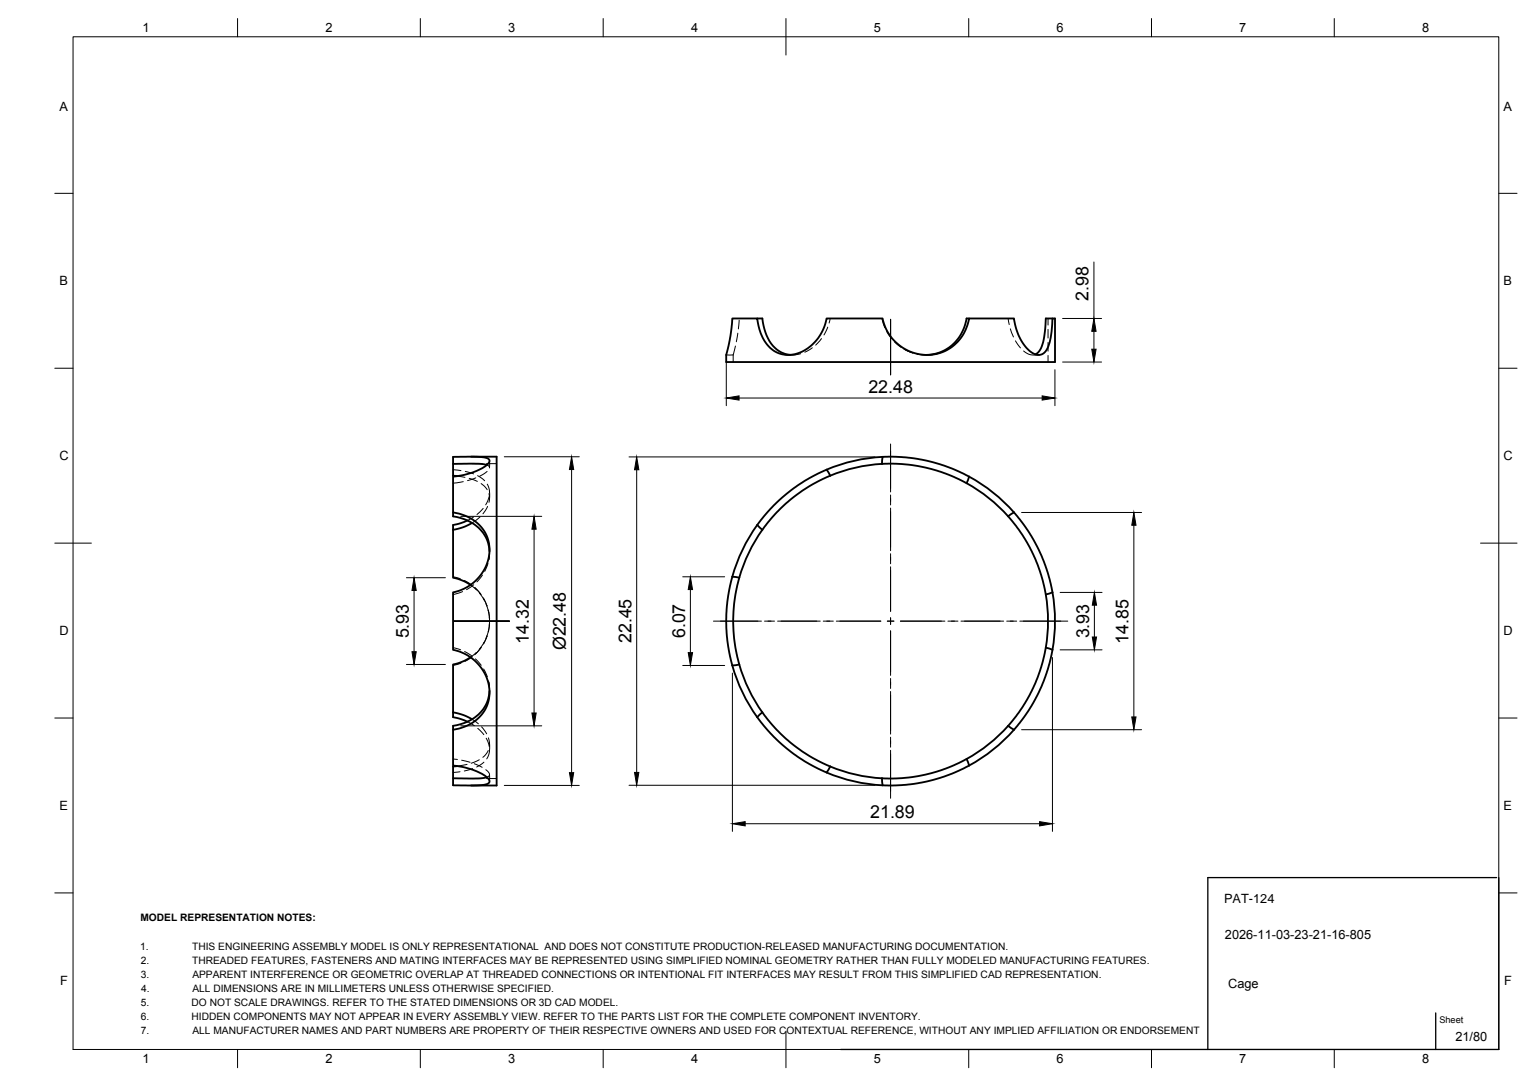
ISO-10303-21;
HEADER;
/* Generated by software containing ST-Developer
 * from STEP Tools, Inc. (www.steptools.com) 
 */

FILE_DESCRIPTION(
/* description */ ('XY cross-slide table'),
/* implementation_level */ '2;1');

FILE_NAME(
/* name */ 'Cage.step',
/* time_stamp */ '2026-10-28T03:22:46-07:00',
/* author */ (''),
/* organization */ (''),
/* preprocessor_version */ 'ST-DEVELOPER v20.2',
/* originating_system */ 'Autodesk Translation Framework v15.17.0.0',
/* authorisation */ '');

FILE_SCHEMA (('AUTOMOTIVE_DESIGN { 1 0 10303 214 3 1 1 }'));
ENDSEC;

DATA;
#10=MECHANICAL_DESIGN_GEOMETRIC_PRESENTATION_REPRESENTATION('',(#1690),#62984);
#693=B_SPLINE_CURVE_WITH_KNOTS('',3,(#33674,#33675,#33676,#33677,#33678,
#33679,#33680,#33681,#33682,#33683,#33684,#33685,#33686,#33687,#33688,#33689,
#33690,#33691,#33692,#33693,#33694,#33695),.UNSPECIFIED.,.F.,.F.,(4,2,2,
2,2,2,2,2,2,2,4),(0.0591825211272536,0.157966726598481,0.236950089897721,
0.315933453196962,0.391576304923761,0.46721915665056,0.54286200837736,0.618504860104159,
0.697488223403399,0.77647158670264,0.875255792173867),.UNSPECIFIED.);
#694=B_SPLINE_CURVE_WITH_KNOTS('',3,(#33699,#33700,#33701,#33702,#33703,
#33704,#33705,#33706,#33707,#33708,#33709,#33710,#33711,#33712,#33713,#33714,
#33715,#33716,#33717,#33718,#33719,#33720),.UNSPECIFIED.,.F.,.F.,(4,2,2,
2,2,2,2,2,2,2,4),(0.0581119756758434,0.106553146291161,0.213106292582322,
0.30849933801665,0.386091982889075,0.4636846277615,0.541277272633925,0.61886991750635,
0.714262962940678,0.820816109231839,0.869257279847157),.UNSPECIFIED.);
#695=B_SPLINE_CURVE_WITH_KNOTS('',3,(#33726,#33727,#33728,#33729,#33730,
#33731,#33732,#33733,#33734,#33735,#33736,#33737,#33738,#33739,#33740,#33741,
#33742,#33743,#33744,#33745,#33746,#33747),.UNSPECIFIED.,.F.,.F.,(4,2,2,
2,2,2,2,2,2,2,4),(0.0581119756758434,0.106553146291161,0.213106292582322,
0.30849933801665,0.386091982889075,0.4636846277615,0.541277272633925,0.61886991750635,
0.714262962940679,0.820816109231839,0.869257279847157),.UNSPECIFIED.);
#696=B_SPLINE_CURVE_WITH_KNOTS('',3,(#33751,#33752,#33753,#33754,#33755,
#33756,#33757,#33758,#33759,#33760,#33761,#33762,#33763,#33764,#33765,#33766,
#33767,#33768,#33769,#33770,#33771,#33772),.UNSPECIFIED.,.F.,.F.,(4,2,2,
2,2,2,2,2,2,2,4),(0.0581119756758433,0.106553146291161,0.213106292582322,
0.308499338016649,0.386091982889075,0.4636846277615,0.541277272633925,0.61886991750635,
0.714262962940678,0.820816109231839,0.869257279847157),.UNSPECIFIED.);
#697=B_SPLINE_CURVE_WITH_KNOTS('',3,(#33781,#33782,#33783,#33784,#33785,
#33786,#33787,#33788,#33789,#33790,#33791,#33792,#33793,#33794,#33795,#33796,
#33797,#33798,#33799,#33800,#33801,#33802),.UNSPECIFIED.,.F.,.F.,(4,2,2,
2,2,2,2,2,2,2,4),(0.0581119756758433,0.106553146291161,0.213106292582322,
0.30849933801665,0.386091982889075,0.4636846277615,0.541277272633925,0.61886991750635,
0.714262962940678,0.820816109231839,0.869257279847157),.UNSPECIFIED.);
#698=B_SPLINE_CURVE_WITH_KNOTS('',3,(#33806,#33807,#33808,#33809,#33810,
#33811,#33812,#33813,#33814,#33815,#33816,#33817,#33818,#33819,#33820,#33821,
#33822,#33823,#33824,#33825,#33826,#33827),.UNSPECIFIED.,.F.,.F.,(4,2,2,
2,2,2,2,2,2,2,4),(0.0581119756758434,0.106553146291161,0.213106292582322,
0.30849933801665,0.386091982889075,0.4636846277615,0.541277272633925,0.61886991750635,
0.714262962940678,0.820816109231839,0.869257279847157),.UNSPECIFIED.);
#699=B_SPLINE_CURVE_WITH_KNOTS('',3,(#33831,#33832,#33833,#33834,#33835,
#33836,#33837,#33838,#33839,#33840,#33841,#33842,#33843,#33844,#33845,#33846,
#33847,#33848,#33849,#33850,#33851,#33852),.UNSPECIFIED.,.F.,.F.,(4,2,2,
2,2,2,2,2,2,2,4),(0.0581119756758434,0.106553146291161,0.213106292582322,
0.30849933801665,0.386091982889075,0.4636846277615,0.541277272633925,0.61886991750635,
0.714262962940678,0.820816109231839,0.869257279847157),.UNSPECIFIED.);
#700=B_SPLINE_CURVE_WITH_KNOTS('',3,(#33856,#33857,#33858,#33859,#33860,
#33861,#33862,#33863,#33864,#33865,#33866,#33867,#33868,#33869,#33870,#33871,
#33872,#33873,#33874,#33875,#33876,#33877),.UNSPECIFIED.,.F.,.F.,(4,2,2,
2,2,2,2,2,2,2,4),(0.0581119756758433,0.106553146291161,0.213106292582322,
0.30849933801665,0.386091982889075,0.4636846277615,0.541277272633925,0.61886991750635,
0.714262962940678,0.820816109231839,0.869257279847157),.UNSPECIFIED.);
#701=B_SPLINE_CURVE_WITH_KNOTS('',3,(#33885,#33886,#33887,#33888,#33889,
#33890,#33891,#33892,#33893,#33894,#33895,#33896,#33897,#33898,#33899,#33900,
#33901,#33902,#33903,#33904,#33905,#33906),.UNSPECIFIED.,.F.,.F.,(4,2,2,
2,2,2,2,2,2,2,4),(0.0591825211272536,0.157966726598481,0.236950089897721,
0.315933453196962,0.391576304923761,0.467219156650561,0.54286200837736,
0.618504860104159,0.697488223403399,0.77647158670264,0.875255792173867),
 .UNSPECIFIED.);
#702=B_SPLINE_CURVE_WITH_KNOTS('',3,(#33914,#33915,#33916,#33917,#33918,
#33919,#33920,#33921,#33922,#33923,#33924,#33925,#33926,#33927,#33928,#33929,
#33930,#33931,#33932,#33933,#33934,#33935),.UNSPECIFIED.,.F.,.F.,(4,2,2,
2,2,2,2,2,2,2,4),(0.0591825211272536,0.157966726598481,0.236950089897722,
0.315933453196962,0.391576304923761,0.467219156650561,0.54286200837736,
0.618504860104159,0.697488223403399,0.77647158670264,0.875255792173867),
 .UNSPECIFIED.);
#703=B_SPLINE_CURVE_WITH_KNOTS('',3,(#33945,#33946,#33947,#33948,#33949,
#33950,#33951,#33952,#33953,#33954,#33955,#33956,#33957,#33958,#33959,#33960,
#33961,#33962,#33963,#33964,#33965,#33966),.UNSPECIFIED.,.F.,.F.,(4,2,2,
2,2,2,2,2,2,2,4),(0.0591825211272536,0.157966726598481,0.236950089897721,
0.315933453196962,0.391576304923761,0.46721915665056,0.54286200837736,0.618504860104159,
0.697488223403399,0.77647158670264,0.875255792173867),.UNSPECIFIED.);
#704=B_SPLINE_CURVE_WITH_KNOTS('',3,(#33974,#33975,#33976,#33977,#33978,
#33979,#33980,#33981,#33982,#33983,#33984,#33985,#33986,#33987,#33988,#33989,
#33990,#33991,#33992,#33993,#33994,#33995),.UNSPECIFIED.,.F.,.F.,(4,2,2,
2,2,2,2,2,2,2,4),(0.0591825211272536,0.157966726598481,0.236950089897721,
0.315933453196962,0.391576304923761,0.46721915665056,0.542862008377359,
0.618504860104159,0.697488223403399,0.776471586702639,0.875255792173867),
 .UNSPECIFIED.);
#705=B_SPLINE_CURVE_WITH_KNOTS('',3,(#34003,#34004,#34005,#34006,#34007,
#34008,#34009,#34010,#34011,#34012,#34013,#34014,#34015,#34016,#34017,#34018,
#34019,#34020,#34021,#34022,#34023,#34024),.UNSPECIFIED.,.F.,.F.,(4,2,2,
2,2,2,2,2,2,2,4),(0.0591825211272536,0.157966726598481,0.236950089897721,
0.315933453196962,0.391576304923761,0.46721915665056,0.54286200837736,0.618504860104159,
0.697488223403399,0.77647158670264,0.875255792173867),.UNSPECIFIED.);
#706=B_SPLINE_CURVE_WITH_KNOTS('',3,(#34033,#34034,#34035,#34036,#34037,
#34038,#34039,#34040,#34041,#34042,#34043,#34044,#34045,#34046,#34047,#34048,
#34049,#34050,#34051,#34052,#34053,#34054),.UNSPECIFIED.,.F.,.F.,(4,2,2,
2,2,2,2,2,2,2,4),(0.0591825211272536,0.157966726598481,0.236950089897721,
0.315933453196962,0.391576304923761,0.46721915665056,0.542862008377359,
0.618504860104159,0.697488223403399,0.776471586702639,0.875255792173867),
 .UNSPECIFIED.);
#1388=SPHERICAL_SURFACE('',#24342,0.309556);
#1389=SPHERICAL_SURFACE('',#24358,0.309556);
#1390=SPHERICAL_SURFACE('',#24363,0.309556);
#1391=SPHERICAL_SURFACE('',#24369,0.309556);
#1392=SPHERICAL_SURFACE('',#24374,0.309556);
#1393=SPHERICAL_SURFACE('',#24379,0.309556);
#1394=SPHERICAL_SURFACE('',#24387,0.309556);
#1518=SHAPE_REPRESENTATION_RELATIONSHIP('SRR','None',#63367,#1601);
#1601=ADVANCED_BREP_SHAPE_REPRESENTATION('',(#1803),#62904);
#1690=STYLED_ITEM('',(#63912),#1803);
#1803=MANIFOLD_SOLID_BREP('Continuous crown cage',#22984);
#1987=FACE_BOUND('',#4469,.T.);
#2385=PLANE('',#24355);
#2386=PLANE('',#24360);
#2387=PLANE('',#24365);
#2388=PLANE('',#24371);
#2389=PLANE('',#24376);
#2390=PLANE('',#24385);
#2391=PLANE('',#24389);
#2392=PLANE('',#24390);
#3039=FACE_OUTER_BOUND('',#4453,.T.);
#3040=FACE_OUTER_BOUND('',#4454,.T.);
#3041=FACE_OUTER_BOUND('',#4455,.T.);
#3042=FACE_OUTER_BOUND('',#4456,.T.);
#3043=FACE_OUTER_BOUND('',#4457,.T.);
#3044=FACE_OUTER_BOUND('',#4458,.T.);
#3045=FACE_OUTER_BOUND('',#4459,.T.);
#3046=FACE_OUTER_BOUND('',#4460,.T.);
#3047=FACE_OUTER_BOUND('',#4461,.T.);
#3048=FACE_OUTER_BOUND('',#4462,.T.);
#3049=FACE_OUTER_BOUND('',#4463,.T.);
#3050=FACE_OUTER_BOUND('',#4464,.T.);
#3051=FACE_OUTER_BOUND('',#4465,.T.);
#3052=FACE_OUTER_BOUND('',#4466,.T.);
#3053=FACE_OUTER_BOUND('',#4467,.T.);
#3054=FACE_OUTER_BOUND('',#4468,.T.);
#3055=FACE_OUTER_BOUND('',#4470,.T.);
#4453=EDGE_LOOP('',(#15632,#15633,#15634,#15635));
#4454=EDGE_LOOP('',(#15636,#15637,#15638,#15639,#15640,#15641,#15642,#15643,
#15644,#15645,#15646,#15647,#15648,#15649,#15650,#15651,#15652,#15653));
#4455=EDGE_LOOP('',(#15654,#15655,#15656,#15657));
#4456=EDGE_LOOP('',(#15658,#15659,#15660,#15661));
#4457=EDGE_LOOP('',(#15662,#15663,#15664,#15665));
#4458=EDGE_LOOP('',(#15666,#15667,#15668,#15669));
#4459=EDGE_LOOP('',(#15670,#15671,#15672,#15673,#15674,#15675));
#4460=EDGE_LOOP('',(#15676,#15677,#15678,#15679));
#4461=EDGE_LOOP('',(#15680,#15681,#15682,#15683));
#4462=EDGE_LOOP('',(#15684,#15685,#15686,#15687));
#4463=EDGE_LOOP('',(#15688,#15689,#15690,#15691));
#4464=EDGE_LOOP('',(#15692,#15693,#15694,#15695));
#4465=EDGE_LOOP('',(#15696,#15697,#15698,#15699,#15700,#15701,#15702,#15703,
#15704,#15705,#15706,#15707,#15708,#15709,#15710,#15711,#15712,#15713));
#4466=EDGE_LOOP('',(#15714,#15715,#15716,#15717));
#4467=EDGE_LOOP('',(#15718,#15719,#15720,#15721));
#4468=EDGE_LOOP('',(#15722));
#4469=EDGE_LOOP('',(#15723));
#4470=EDGE_LOOP('',(#15724,#15725,#15726,#15727));
#6117=LINE('',#33776,#7604);
#6118=LINE('',#34029,#7605);
#7604=VECTOR('',#27370,1.123812);
#7605=VECTOR('',#27439,1.076188);
#9033=CIRCLE('',#24343,0.303778037777585);
#9034=CIRCLE('',#24344,0.303778037777585);
#9035=CIRCLE('',#24346,1.123812);
#9036=CIRCLE('',#24347,1.123812);
#9037=CIRCLE('',#24348,1.123812);
#9038=CIRCLE('',#24349,1.123812);
#9039=CIRCLE('',#24350,1.123812);
#9040=CIRCLE('',#24351,1.123812);
#9041=CIRCLE('',#24352,1.123812);
#9042=CIRCLE('',#24353,1.123812);
#9043=CIRCLE('',#24354,1.123812);
#9044=CIRCLE('',#24356,1.076188);
#9045=CIRCLE('',#24357,0.303778037777585);
#9046=CIRCLE('',#24359,0.303778037777585);
#9047=CIRCLE('',#24361,1.076188);
#9048=CIRCLE('',#24362,0.303778037777585);
#9049=CIRCLE('',#24364,0.303778037777585);
#9050=CIRCLE('',#24366,1.076188);
#9051=CIRCLE('',#24367,1.076188);
#9052=CIRCLE('',#24368,0.303778037777585);
#9053=CIRCLE('',#24370,0.303778037777585);
#9054=CIRCLE('',#24372,1.076188);
#9055=CIRCLE('',#24373,0.303778037777585);
#9056=CIRCLE('',#24375,0.303778037777585);
#9057=CIRCLE('',#24377,1.076188);
#9058=CIRCLE('',#24378,0.303778037777585);
#9059=CIRCLE('',#24380,0.303778037777585);
#9060=CIRCLE('',#24382,1.076188);
#9061=CIRCLE('',#24383,1.076188);
#9062=CIRCLE('',#24384,1.076188);
#9063=CIRCLE('',#24386,0.303778037777585);
#9064=CIRCLE('',#24388,0.303778037777585);
#10021=VERTEX_POINT('',#33672);
#10022=VERTEX_POINT('',#33673);
#10023=VERTEX_POINT('',#33696);
#10024=VERTEX_POINT('',#33698);
#10025=VERTEX_POINT('',#33723);
#10026=VERTEX_POINT('',#33725);
#10027=VERTEX_POINT('',#33748);
#10028=VERTEX_POINT('',#33750);
#10029=VERTEX_POINT('',#33773);
#10030=VERTEX_POINT('',#33775);
#10031=VERTEX_POINT('',#33778);
#10032=VERTEX_POINT('',#33780);
#10033=VERTEX_POINT('',#33803);
#10034=VERTEX_POINT('',#33805);
#10035=VERTEX_POINT('',#33828);
#10036=VERTEX_POINT('',#33830);
#10037=VERTEX_POINT('',#33853);
#10038=VERTEX_POINT('',#33855);
#10039=VERTEX_POINT('',#33880);
#10040=VERTEX_POINT('',#33884);
#10041=VERTEX_POINT('',#33909);
#10042=VERTEX_POINT('',#33913);
#10043=VERTEX_POINT('',#33938);
#10044=VERTEX_POINT('',#33940);
#10045=VERTEX_POINT('',#33944);
#10046=VERTEX_POINT('',#33969);
#10047=VERTEX_POINT('',#33973);
#10048=VERTEX_POINT('',#33998);
#10049=VERTEX_POINT('',#34002);
#10050=VERTEX_POINT('',#34027);
#10051=VERTEX_POINT('',#34030);
#10052=VERTEX_POINT('',#34032);
#12200=EDGE_CURVE('',#10021,#10022,#693,.T.);
#12201=EDGE_CURVE('',#10023,#10021,#9033,.T.);
#12202=EDGE_CURVE('',#10024,#10023,#694,.T.);
#12203=EDGE_CURVE('',#10022,#10024,#9034,.T.);
#12204=EDGE_CURVE('',#10025,#10023,#9035,.T.);
#12205=EDGE_CURVE('',#10025,#10026,#695,.T.);
#12206=EDGE_CURVE('',#10027,#10026,#9036,.T.);
#12207=EDGE_CURVE('',#10027,#10028,#696,.T.);
#12208=EDGE_CURVE('',#10029,#10028,#9037,.T.);
#12209=EDGE_CURVE('',#10029,#10030,#6117,.T.);
#12210=EDGE_CURVE('',#10030,#10030,#9038,.T.);
#12211=EDGE_CURVE('',#10031,#10029,#9039,.T.);
#12212=EDGE_CURVE('',#10031,#10032,#697,.T.);
#12213=EDGE_CURVE('',#10033,#10032,#9040,.T.);
#12214=EDGE_CURVE('',#10033,#10034,#698,.T.);
#12215=EDGE_CURVE('',#10035,#10034,#9041,.T.);
#12216=EDGE_CURVE('',#10035,#10036,#699,.T.);
#12217=EDGE_CURVE('',#10037,#10036,#9042,.T.);
#12218=EDGE_CURVE('',#10037,#10038,#700,.T.);
#12219=EDGE_CURVE('',#10024,#10038,#9043,.T.);
#12220=EDGE_CURVE('',#10021,#10039,#9044,.T.);
#12221=EDGE_CURVE('',#10039,#10025,#9045,.T.);
#12222=EDGE_CURVE('',#10040,#10039,#701,.T.);
#12223=EDGE_CURVE('',#10026,#10040,#9046,.T.);
#12224=EDGE_CURVE('',#10040,#10041,#9047,.T.);
#12225=EDGE_CURVE('',#10041,#10027,#9048,.T.);
#12226=EDGE_CURVE('',#10042,#10041,#702,.T.);
#12227=EDGE_CURVE('',#10028,#10042,#9049,.T.);
#12228=EDGE_CURVE('',#10042,#10043,#9050,.T.);
#12229=EDGE_CURVE('',#10043,#10044,#9051,.T.);
#12230=EDGE_CURVE('',#10044,#10031,#9052,.T.);
#12231=EDGE_CURVE('',#10045,#10044,#703,.T.);
#12232=EDGE_CURVE('',#10032,#10045,#9053,.T.);
#12233=EDGE_CURVE('',#10045,#10046,#9054,.T.);
#12234=EDGE_CURVE('',#10046,#10033,#9055,.T.);
#12235=EDGE_CURVE('',#10047,#10046,#704,.T.);
#12236=EDGE_CURVE('',#10034,#10047,#9056,.T.);
#12237=EDGE_CURVE('',#10047,#10048,#9057,.T.);
#12238=EDGE_CURVE('',#10048,#10035,#9058,.T.);
#12239=EDGE_CURVE('',#10049,#10048,#705,.T.);
#12240=EDGE_CURVE('',#10036,#10049,#9059,.T.);
#12241=EDGE_CURVE('',#10050,#10050,#9060,.T.);
#12242=EDGE_CURVE('',#10050,#10043,#6118,.T.);
#12243=EDGE_CURVE('',#10051,#10022,#9061,.T.);
#12244=EDGE_CURVE('',#10051,#10052,#706,.T.);
#12245=EDGE_CURVE('',#10049,#10052,#9062,.T.);
#12246=EDGE_CURVE('',#10038,#10051,#9063,.T.);
#12247=EDGE_CURVE('',#10052,#10037,#9064,.T.);
#15632=ORIENTED_EDGE('',*,*,#12200,.F.);
#15633=ORIENTED_EDGE('',*,*,#12201,.F.);
#15634=ORIENTED_EDGE('',*,*,#12202,.F.);
#15635=ORIENTED_EDGE('',*,*,#12203,.F.);
#15636=ORIENTED_EDGE('',*,*,#12202,.T.);
#15637=ORIENTED_EDGE('',*,*,#12204,.F.);
#15638=ORIENTED_EDGE('',*,*,#12205,.T.);
#15639=ORIENTED_EDGE('',*,*,#12206,.F.);
#15640=ORIENTED_EDGE('',*,*,#12207,.T.);
#15641=ORIENTED_EDGE('',*,*,#12208,.F.);
#15642=ORIENTED_EDGE('',*,*,#12209,.T.);
#15643=ORIENTED_EDGE('',*,*,#12210,.F.);
#15644=ORIENTED_EDGE('',*,*,#12209,.F.);
#15645=ORIENTED_EDGE('',*,*,#12211,.F.);
#15646=ORIENTED_EDGE('',*,*,#12212,.T.);
#15647=ORIENTED_EDGE('',*,*,#12213,.F.);
#15648=ORIENTED_EDGE('',*,*,#12214,.T.);
#15649=ORIENTED_EDGE('',*,*,#12215,.F.);
#15650=ORIENTED_EDGE('',*,*,#12216,.T.);
#15651=ORIENTED_EDGE('',*,*,#12217,.F.);
#15652=ORIENTED_EDGE('',*,*,#12218,.T.);
#15653=ORIENTED_EDGE('',*,*,#12219,.F.);
#15654=ORIENTED_EDGE('',*,*,#12201,.T.);
#15655=ORIENTED_EDGE('',*,*,#12220,.T.);
#15656=ORIENTED_EDGE('',*,*,#12221,.T.);
#15657=ORIENTED_EDGE('',*,*,#12204,.T.);
#15658=ORIENTED_EDGE('',*,*,#12222,.F.);
#15659=ORIENTED_EDGE('',*,*,#12223,.F.);
#15660=ORIENTED_EDGE('',*,*,#12205,.F.);
#15661=ORIENTED_EDGE('',*,*,#12221,.F.);
#15662=ORIENTED_EDGE('',*,*,#12223,.T.);
#15663=ORIENTED_EDGE('',*,*,#12224,.T.);
#15664=ORIENTED_EDGE('',*,*,#12225,.T.);
#15665=ORIENTED_EDGE('',*,*,#12206,.T.);
#15666=ORIENTED_EDGE('',*,*,#12226,.F.);
#15667=ORIENTED_EDGE('',*,*,#12227,.F.);
#15668=ORIENTED_EDGE('',*,*,#12207,.F.);
#15669=ORIENTED_EDGE('',*,*,#12225,.F.);
#15670=ORIENTED_EDGE('',*,*,#12227,.T.);
#15671=ORIENTED_EDGE('',*,*,#12228,.T.);
#15672=ORIENTED_EDGE('',*,*,#12229,.T.);
#15673=ORIENTED_EDGE('',*,*,#12230,.T.);
#15674=ORIENTED_EDGE('',*,*,#12211,.T.);
#15675=ORIENTED_EDGE('',*,*,#12208,.T.);
#15676=ORIENTED_EDGE('',*,*,#12231,.F.);
#15677=ORIENTED_EDGE('',*,*,#12232,.F.);
#15678=ORIENTED_EDGE('',*,*,#12212,.F.);
#15679=ORIENTED_EDGE('',*,*,#12230,.F.);
#15680=ORIENTED_EDGE('',*,*,#12232,.T.);
#15681=ORIENTED_EDGE('',*,*,#12233,.T.);
#15682=ORIENTED_EDGE('',*,*,#12234,.T.);
#15683=ORIENTED_EDGE('',*,*,#12213,.T.);
#15684=ORIENTED_EDGE('',*,*,#12235,.F.);
#15685=ORIENTED_EDGE('',*,*,#12236,.F.);
#15686=ORIENTED_EDGE('',*,*,#12214,.F.);
#15687=ORIENTED_EDGE('',*,*,#12234,.F.);
#15688=ORIENTED_EDGE('',*,*,#12236,.T.);
#15689=ORIENTED_EDGE('',*,*,#12237,.T.);
#15690=ORIENTED_EDGE('',*,*,#12238,.T.);
#15691=ORIENTED_EDGE('',*,*,#12215,.T.);
#15692=ORIENTED_EDGE('',*,*,#12216,.F.);
#15693=ORIENTED_EDGE('',*,*,#12238,.F.);
#15694=ORIENTED_EDGE('',*,*,#12239,.F.);
#15695=ORIENTED_EDGE('',*,*,#12240,.F.);
#15696=ORIENTED_EDGE('',*,*,#12241,.F.);
#15697=ORIENTED_EDGE('',*,*,#12242,.T.);
#15698=ORIENTED_EDGE('',*,*,#12228,.F.);
#15699=ORIENTED_EDGE('',*,*,#12226,.T.);
#15700=ORIENTED_EDGE('',*,*,#12224,.F.);
#15701=ORIENTED_EDGE('',*,*,#12222,.T.);
#15702=ORIENTED_EDGE('',*,*,#12220,.F.);
#15703=ORIENTED_EDGE('',*,*,#12200,.T.);
#15704=ORIENTED_EDGE('',*,*,#12243,.F.);
#15705=ORIENTED_EDGE('',*,*,#12244,.T.);
#15706=ORIENTED_EDGE('',*,*,#12245,.F.);
#15707=ORIENTED_EDGE('',*,*,#12239,.T.);
#15708=ORIENTED_EDGE('',*,*,#12237,.F.);
#15709=ORIENTED_EDGE('',*,*,#12235,.T.);
#15710=ORIENTED_EDGE('',*,*,#12233,.F.);
#15711=ORIENTED_EDGE('',*,*,#12231,.T.);
#15712=ORIENTED_EDGE('',*,*,#12229,.F.);
#15713=ORIENTED_EDGE('',*,*,#12242,.F.);
#15714=ORIENTED_EDGE('',*,*,#12203,.T.);
#15715=ORIENTED_EDGE('',*,*,#12219,.T.);
#15716=ORIENTED_EDGE('',*,*,#12246,.T.);
#15717=ORIENTED_EDGE('',*,*,#12243,.T.);
#15718=ORIENTED_EDGE('',*,*,#12218,.F.);
#15719=ORIENTED_EDGE('',*,*,#12247,.F.);
#15720=ORIENTED_EDGE('',*,*,#12244,.F.);
#15721=ORIENTED_EDGE('',*,*,#12246,.F.);
#15722=ORIENTED_EDGE('',*,*,#12210,.T.);
#15723=ORIENTED_EDGE('',*,*,#12241,.T.);
#15724=ORIENTED_EDGE('',*,*,#12240,.T.);
#15725=ORIENTED_EDGE('',*,*,#12245,.T.);
#15726=ORIENTED_EDGE('',*,*,#12247,.T.);
#15727=ORIENTED_EDGE('',*,*,#12217,.T.);
#21108=CYLINDRICAL_SURFACE('',#24345,1.123812);
#21109=CYLINDRICAL_SURFACE('',#24381,1.076188);
#21820=ADVANCED_FACE('',(#3039),#1388,.F.);
#21821=ADVANCED_FACE('',(#3040),#21108,.T.);
#21822=ADVANCED_FACE('',(#3041),#2385,.T.);
#21823=ADVANCED_FACE('',(#3042),#1389,.F.);
#21824=ADVANCED_FACE('',(#3043),#2386,.T.);
#21825=ADVANCED_FACE('',(#3044),#1390,.F.);
#21826=ADVANCED_FACE('',(#3045),#2387,.T.);
#21827=ADVANCED_FACE('',(#3046),#1391,.F.);
#21828=ADVANCED_FACE('',(#3047),#2388,.T.);
#21829=ADVANCED_FACE('',(#3048),#1392,.F.);
#21830=ADVANCED_FACE('',(#3049),#2389,.T.);
#21831=ADVANCED_FACE('',(#3050),#1393,.F.);
#21832=ADVANCED_FACE('',(#3051),#21109,.F.);
#21833=ADVANCED_FACE('',(#3052),#2390,.T.);
#21834=ADVANCED_FACE('',(#3053),#1394,.F.);
#21835=ADVANCED_FACE('',(#3054,#1987),#2391,.T.);
#21836=ADVANCED_FACE('',(#3055),#2392,.T.);
#22984=CLOSED_SHELL('',(#21820,#21821,#21822,#21823,#21824,#21825,#21826,
#21827,#21828,#21829,#21830,#21831,#21832,#21833,#21834,#21835,#21836));
#24341=AXIS2_PLACEMENT_3D('',#33670,#27354,#27355);
#24342=AXIS2_PLACEMENT_3D('',#33671,#27356,#27357);
#24343=AXIS2_PLACEMENT_3D('',#33697,#27358,#27359);
#24344=AXIS2_PLACEMENT_3D('',#33721,#27360,#27361);
#24345=AXIS2_PLACEMENT_3D('',#33722,#27362,#27363);
#24346=AXIS2_PLACEMENT_3D('',#33724,#27364,#27365);
#24347=AXIS2_PLACEMENT_3D('',#33749,#27366,#27367);
#24348=AXIS2_PLACEMENT_3D('',#33774,#27368,#27369);
#24349=AXIS2_PLACEMENT_3D('',#33777,#27371,#27372);
#24350=AXIS2_PLACEMENT_3D('',#33779,#27373,#27374);
#24351=AXIS2_PLACEMENT_3D('',#33804,#27375,#27376);
#24352=AXIS2_PLACEMENT_3D('',#33829,#27377,#27378);
#24353=AXIS2_PLACEMENT_3D('',#33854,#27379,#27380);
#24354=AXIS2_PLACEMENT_3D('',#33878,#27381,#27382);
#24355=AXIS2_PLACEMENT_3D('',#33879,#27383,#27384);
#24356=AXIS2_PLACEMENT_3D('',#33881,#27385,#27386);
#24357=AXIS2_PLACEMENT_3D('',#33882,#27387,#27388);
#24358=AXIS2_PLACEMENT_3D('',#33883,#27389,#27390);
#24359=AXIS2_PLACEMENT_3D('',#33907,#27391,#27392);
#24360=AXIS2_PLACEMENT_3D('',#33908,#27393,#27394);
#24361=AXIS2_PLACEMENT_3D('',#33910,#27395,#27396);
#24362=AXIS2_PLACEMENT_3D('',#33911,#27397,#27398);
#24363=AXIS2_PLACEMENT_3D('',#33912,#27399,#27400);
#24364=AXIS2_PLACEMENT_3D('',#33936,#27401,#27402);
#24365=AXIS2_PLACEMENT_3D('',#33937,#27403,#27404);
#24366=AXIS2_PLACEMENT_3D('',#33939,#27405,#27406);
#24367=AXIS2_PLACEMENT_3D('',#33941,#27407,#27408);
#24368=AXIS2_PLACEMENT_3D('',#33942,#27409,#27410);
#24369=AXIS2_PLACEMENT_3D('',#33943,#27411,#27412);
#24370=AXIS2_PLACEMENT_3D('',#33967,#27413,#27414);
#24371=AXIS2_PLACEMENT_3D('',#33968,#27415,#27416);
#24372=AXIS2_PLACEMENT_3D('',#33970,#27417,#27418);
#24373=AXIS2_PLACEMENT_3D('',#33971,#27419,#27420);
#24374=AXIS2_PLACEMENT_3D('',#33972,#27421,#27422);
#24375=AXIS2_PLACEMENT_3D('',#33996,#27423,#27424);
#24376=AXIS2_PLACEMENT_3D('',#33997,#27425,#27426);
#24377=AXIS2_PLACEMENT_3D('',#33999,#27427,#27428);
#24378=AXIS2_PLACEMENT_3D('',#34000,#27429,#27430);
#24379=AXIS2_PLACEMENT_3D('',#34001,#27431,#27432);
#24380=AXIS2_PLACEMENT_3D('',#34025,#27433,#27434);
#24381=AXIS2_PLACEMENT_3D('',#34026,#27435,#27436);
#24382=AXIS2_PLACEMENT_3D('',#34028,#27437,#27438);
#24383=AXIS2_PLACEMENT_3D('',#34031,#27440,#27441);
#24384=AXIS2_PLACEMENT_3D('',#34055,#27442,#27443);
#24385=AXIS2_PLACEMENT_3D('',#34056,#27444,#27445);
#24386=AXIS2_PLACEMENT_3D('',#34057,#27446,#27447);
#24387=AXIS2_PLACEMENT_3D('',#34058,#27448,#27449);
#24388=AXIS2_PLACEMENT_3D('',#34059,#27450,#27451);
#24389=AXIS2_PLACEMENT_3D('',#34060,#27452,#27453);
#24390=AXIS2_PLACEMENT_3D('',#34061,#27454,#27455);
#27354=DIRECTION('axis',(0.,0.,1.));
#27355=DIRECTION('refdir',(1.,0.,0.));
#27356=DIRECTION('center_axis',(0.,0.,1.));
#27357=DIRECTION('ref_axis',(1.,0.,0.));
#27358=DIRECTION('center_axis',(0.,-1.,0.));
#27359=DIRECTION('ref_axis',(0.,0.,-1.));
#27360=DIRECTION('center_axis',(0.,-1.,0.));
#27361=DIRECTION('ref_axis',(0.,0.,-1.));
#27362=DIRECTION('center_axis',(0.,1.,0.));
#27363=DIRECTION('ref_axis',(1.,0.,0.));
#27364=DIRECTION('center_axis',(0.,1.,0.));
#27365=DIRECTION('ref_axis',(1.,0.,0.));
#27366=DIRECTION('center_axis',(0.,1.,0.));
#27367=DIRECTION('ref_axis',(1.,0.,0.));
#27368=DIRECTION('center_axis',(0.,1.,0.));
#27369=DIRECTION('ref_axis',(1.,0.,0.));
#27370=DIRECTION('',(0.,-1.,0.));
#27371=DIRECTION('center_axis',(0.,-1.,0.));
#27372=DIRECTION('ref_axis',(1.,0.,0.));
#27373=DIRECTION('center_axis',(0.,1.,0.));
#27374=DIRECTION('ref_axis',(1.,0.,0.));
#27375=DIRECTION('center_axis',(0.,1.,0.));
#27376=DIRECTION('ref_axis',(1.,0.,0.));
#27377=DIRECTION('center_axis',(0.,1.,0.));
#27378=DIRECTION('ref_axis',(1.,0.,0.));
#27379=DIRECTION('center_axis',(0.,1.,0.));
#27380=DIRECTION('ref_axis',(1.,0.,0.));
#27381=DIRECTION('center_axis',(0.,1.,0.));
#27382=DIRECTION('ref_axis',(1.,0.,0.));
#27383=DIRECTION('center_axis',(0.,1.,0.));
#27384=DIRECTION('ref_axis',(1.,0.,0.));
#27385=DIRECTION('center_axis',(0.,-1.,0.));
#27386=DIRECTION('ref_axis',(1.,0.,0.));
#27387=DIRECTION('center_axis',(0.,-1.,0.));
#27388=DIRECTION('ref_axis',(0.,0.,-1.));
#27389=DIRECTION('center_axis',(8.96625347776458E-17,0.,1.));
#27390=DIRECTION('ref_axis',(1.,0.,0.));
#27391=DIRECTION('center_axis',(0.,-1.,0.));
#27392=DIRECTION('ref_axis',(0.,0.,-1.));
#27393=DIRECTION('center_axis',(0.,1.,0.));
#27394=DIRECTION('ref_axis',(1.,0.,0.));
#27395=DIRECTION('center_axis',(0.,-1.,0.));
#27396=DIRECTION('ref_axis',(1.,0.,0.));
#27397=DIRECTION('center_axis',(0.,-1.,0.));
#27398=DIRECTION('ref_axis',(0.,0.,-1.));
#27399=DIRECTION('center_axis',(0.,0.,1.));
#27400=DIRECTION('ref_axis',(1.,0.,0.));
#27401=DIRECTION('center_axis',(0.,-1.,0.));
#27402=DIRECTION('ref_axis',(0.,0.,-1.));
#27403=DIRECTION('center_axis',(0.,1.,0.));
#27404=DIRECTION('ref_axis',(1.,0.,0.));
#27405=DIRECTION('center_axis',(0.,-1.,0.));
#27406=DIRECTION('ref_axis',(1.,0.,0.));
#27407=DIRECTION('center_axis',(0.,-1.,0.));
#27408=DIRECTION('ref_axis',(1.,0.,0.));
#27409=DIRECTION('center_axis',(0.,-1.,0.));
#27410=DIRECTION('ref_axis',(0.,0.,-1.));
#27411=DIRECTION('center_axis',(0.,0.,1.));
#27412=DIRECTION('ref_axis',(1.,0.,0.));
#27413=DIRECTION('center_axis',(0.,-1.,0.));
#27414=DIRECTION('ref_axis',(0.,0.,-1.));
#27415=DIRECTION('center_axis',(0.,1.,0.));
#27416=DIRECTION('ref_axis',(1.,0.,0.));
#27417=DIRECTION('center_axis',(0.,-1.,0.));
#27418=DIRECTION('ref_axis',(1.,0.,0.));
#27419=DIRECTION('center_axis',(0.,-1.,0.));
#27420=DIRECTION('ref_axis',(0.,0.,-1.));
#27421=DIRECTION('center_axis',(8.96625347776458E-17,0.,1.));
#27422=DIRECTION('ref_axis',(1.,0.,0.));
#27423=DIRECTION('center_axis',(0.,-1.,0.));
#27424=DIRECTION('ref_axis',(0.,0.,-1.));
#27425=DIRECTION('center_axis',(0.,1.,0.));
#27426=DIRECTION('ref_axis',(1.,0.,0.));
#27427=DIRECTION('center_axis',(0.,-1.,0.));
#27428=DIRECTION('ref_axis',(1.,0.,0.));
#27429=DIRECTION('center_axis',(0.,-1.,0.));
#27430=DIRECTION('ref_axis',(0.,0.,-1.));
#27431=DIRECTION('center_axis',(0.,0.,1.));
#27432=DIRECTION('ref_axis',(1.,0.,0.));
#27433=DIRECTION('center_axis',(0.,-1.,0.));
#27434=DIRECTION('ref_axis',(0.,0.,-1.));
#27435=DIRECTION('center_axis',(0.,1.,0.));
#27436=DIRECTION('ref_axis',(1.,0.,0.));
#27437=DIRECTION('center_axis',(0.,1.,0.));
#27438=DIRECTION('ref_axis',(1.,0.,0.));
#27439=DIRECTION('',(0.,1.,0.));
#27440=DIRECTION('center_axis',(0.,-1.,0.));
#27441=DIRECTION('ref_axis',(1.,0.,0.));
#27442=DIRECTION('center_axis',(0.,-1.,0.));
#27443=DIRECTION('ref_axis',(1.,0.,0.));
#27444=DIRECTION('center_axis',(0.,1.,0.));
#27445=DIRECTION('ref_axis',(1.,0.,0.));
#27446=DIRECTION('center_axis',(0.,-1.,0.));
#27447=DIRECTION('ref_axis',(0.,0.,-1.));
#27448=DIRECTION('center_axis',(0.,0.,1.));
#27449=DIRECTION('ref_axis',(1.,0.,0.));
#27450=DIRECTION('center_axis',(0.,-1.,0.));
#27451=DIRECTION('ref_axis',(0.,0.,-1.));
#27452=DIRECTION('center_axis',(0.,-1.,0.));
#27453=DIRECTION('ref_axis',(-1.,0.,0.));
#27454=DIRECTION('center_axis',(0.,1.,0.));
#27455=DIRECTION('ref_axis',(1.,0.,0.));
#33670=CARTESIAN_POINT('',(0.,0.,0.));
#33671=CARTESIAN_POINT('Origin',(0.685838782044607,0.,0.860014630714833));
#33672=CARTESIAN_POINT('',(0.413083465285518,-0.05953,0.993751811093549));
#33673=CARTESIAN_POINT('',(0.876916659919095,-0.05953,0.623857181492959));
#33674=CARTESIAN_POINT('Ctrl Pts',(0.413083465285518,-0.05953,0.993751811093549));
#33675=CARTESIAN_POINT('Ctrl Pts',(0.419070565453383,-0.0925528133349865,
0.991263089003441));
#33676=CARTESIAN_POINT('Ctrl Pts',(0.430199341854858,-0.124911173756694,
0.986608710139579));
#33677=CARTESIAN_POINT('Ctrl Pts',(0.457978755888596,-0.177924977804098,
0.973971221090534));
#33678=CARTESIAN_POINT('Ctrl Pts',(0.473077587363685,-0.199697230012983,
0.966820759530997));
#33679=CARTESIAN_POINT('Ctrl Pts',(0.507057380724533,-0.237895043532788,
0.949440676105255));
#33680=CARTESIAN_POINT('Ctrl Pts',(0.525933334162555,-0.254319232363049,
0.939198248544428));
#33681=CARTESIAN_POINT('Ctrl Pts',(0.564362943424238,-0.28018331644634,
0.916597376014514));
#33682=CARTESIAN_POINT('Ctrl Pts',(0.585840553788742,-0.29104845371857,
0.903141581680914));
#33683=CARTESIAN_POINT('Ctrl Pts',(0.629305439856167,-0.30527573347708,
0.873412008702649));
#33684=CARTESIAN_POINT('Ctrl Pts',(0.651278921914856,-0.308638795020976,
0.857118508332695));
#33685=CARTESIAN_POINT('Ctrl Pts',(0.690705563850638,-0.308638795020976,
0.825676810575914));
#33686=CARTESIAN_POINT('Ctrl Pts',(0.711480111898423,-0.30527573347708,
0.807879894508811));
#33687=CARTESIAN_POINT('Ctrl Pts',(0.750136149454208,-0.29104845371857,
0.772120216227122));
#33688=CARTESIAN_POINT('Ctrl Pts',(0.768033796848072,-0.28018331644634,
0.754175290318038));
#33689=CARTESIAN_POINT('Ctrl Pts',(0.798619410861634,-0.254319232363049,
0.721738358858166));
#33690=CARTESIAN_POINT('Ctrl Pts',(0.812805334167529,-0.237895043532788,
0.705614819529209));
#33691=CARTESIAN_POINT('Ctrl Pts',(0.837310877969633,-0.199697230012983,
0.676354402927683));
#33692=CARTESIAN_POINT('Ctrl Pts',(0.847641868610495,-0.177924977804098,
0.663225258065736));
#33693=CARTESIAN_POINT('Ctrl Pts',(0.866144010579847,-0.124911173756694,
0.638954437806245));
#33694=CARTESIAN_POINT('Ctrl Pts',(0.873158080166742,-0.0925528133349865,
0.62914037979579));
#33695=CARTESIAN_POINT('Ctrl Pts',(0.876916659919095,-0.05953,0.623857181492959));
#33696=CARTESIAN_POINT('',(0.437601487681057,-0.05953,1.03511272300331));
#33697=CARTESIAN_POINT('Origin',(0.685838782044607,-0.05953,0.860014630714833));
#33698=CARTESIAN_POINT('',(0.911784794170997,-0.05953,0.656964154625313));
#33699=CARTESIAN_POINT('Ctrl Pts',(0.911784794170998,-0.0595300000000001,
0.656964154625312));
#33700=CARTESIAN_POINT('Ctrl Pts',(0.909827729890942,-0.0762225747374255,
0.659680317203144));
#33701=CARTESIAN_POINT('Ctrl Pts',(0.907004864562642,-0.0928409665394228,
0.663576540841106));
#33702=CARTESIAN_POINT('Ctrl Pts',(0.895234408667242,-0.144299303100741,
0.679480524217551));
#33703=CARTESIAN_POINT('Ctrl Pts',(0.882797231409153,-0.177024326825049,
0.695831250979106));
#33704=CARTESIAN_POINT('Ctrl Pts',(0.854332839576145,-0.227269801620064,
0.73042219438957));
#33705=CARTESIAN_POINT('Ctrl Pts',(0.834863020612702,-0.251265615809407,
0.752807465209441));
#33706=CARTESIAN_POINT('Ctrl Pts',(0.800439809856111,-0.279889827963178,
0.789147407129766));
#33707=CARTESIAN_POINT('Ctrl Pts',(0.781998747691871,-0.290879136862659,
0.80756613568454));
#33708=CARTESIAN_POINT('Ctrl Pts',(0.742239891936898,-0.305251990234487,
0.844254137480382));
#33709=CARTESIAN_POINT('Ctrl Pts',(0.720906778729541,-0.308638795020976,
0.862505527716294));
#33710=CARTESIAN_POINT('Ctrl Pts',(0.680463863683392,-0.308638795020976,
0.894757676234429));
#33711=CARTESIAN_POINT('Ctrl Pts',(0.657923009631182,-0.305251990234488,
0.91149460735272));
#33712=CARTESIAN_POINT('Ctrl Pts',(0.613307674922609,-0.290879136862659,
0.942092777160053));
#33713=CARTESIAN_POINT('Ctrl Pts',(0.591247219971725,-0.279889827963178,
0.955972930713954));
#33714=CARTESIAN_POINT('Ctrl Pts',(0.548158511259202,-0.251265615809407,
0.981446681891443));
#33715=CARTESIAN_POINT('Ctrl Pts',(0.522002043615455,-0.227269801620063,
0.995447160474328));
#33716=CARTESIAN_POINT('Ctrl Pts',(0.481944444320713,-0.177024326825049,
1.01550068154148));
#33717=CARTESIAN_POINT('Ctrl Pts',(0.463236132117164,-0.14429930310074,
1.0239876538093));
#33718=CARTESIAN_POINT('Ctrl Pts',(0.445111721969657,-0.0928409665394226,
1.03192403056628));
#33719=CARTESIAN_POINT('Ctrl Pts',(0.440685038163619,-0.0762225747374254,
1.03380912944435));
#33720=CARTESIAN_POINT('Ctrl Pts',(0.437601487681056,-0.05953,1.03511272300331));
#33721=CARTESIAN_POINT('Origin',(0.685838782044607,-0.05953,0.860014630714833));
#33722=CARTESIAN_POINT('Origin',(0.,-0.208355,0.));
#33723=CARTESIAN_POINT('',(0.0548532617164168,-0.05953,1.12247250791415));
#33724=CARTESIAN_POINT('Origin',(0.,-0.05953,0.));
#33725=CARTESIAN_POINT('',(-0.536443649899848,-0.05953,0.987512846410683));
#33726=CARTESIAN_POINT('Ctrl Pts',(0.0548532617164173,-0.0595300000000001,
1.12247250791414));
#33727=CARTESIAN_POINT('Ctrl Pts',(0.05150947068137,-0.0762225747374254,
1.12263591311425));
#33728=CARTESIAN_POINT('Ctrl Pts',(0.0467032526342597,-0.0928409665394227,
1.12285816383385));
#33729=CARTESIAN_POINT('Ctrl Pts',(0.0269302585198975,-0.144299303100741,
1.12357162229597));
#33730=CARTESIAN_POINT('Ctrl Pts',(0.006392292392153,-0.177024326825049,
1.12404235695137));
#33731=CARTESIAN_POINT('Ctrl Pts',(-0.0383992541984087,-0.227269801620063,
1.12335509974011));
#33732=CARTESIAN_POINT('Ctrl Pts',(-0.0680399972366993,-0.251265615809407,
1.12208997038458));
#33733=CARTESIAN_POINT('Ctrl Pts',(-0.117914228755037,-0.279889827963178,
1.1178344036749));
#33734=CARTESIAN_POINT('Ctrl Pts',(-0.14381238480104,-0.290879136862659,
1.11490049012186));
#33735=CARTESIAN_POINT('Ctrl Pts',(-0.19728546073067,-0.305251990234488,
1.10669035995599));
#33736=CARTESIAN_POINT('Ctrl Pts',(-0.224855950742601,-0.308638795020976,
1.10139101611326));
#33737=CARTESIAN_POINT('Ctrl Pts',(-0.275287440920027,-0.308638795020976,
1.0898803575765));
#33738=CARTESIAN_POINT('Ctrl Pts',(-0.302426893214945,-0.305251990234488,
1.08269251410343));
#33739=CARTESIAN_POINT('Ctrl Pts',(-0.35416671187353,-0.290879136862659,
1.06688848765783));
#33740=CARTESIAN_POINT('Ctrl Pts',(-0.3787731215897,-0.279889827963178,
1.05829506364875));
#33741=CARTESIAN_POINT('Ctrl Pts',(-0.425554672694338,-0.251265615809407,
1.04048957871266));
#33742=CARTESIAN_POINT('Ctrl Pts',(-0.452808978448581,-0.227269801620063,
1.02876878445619));
#33743=CARTESIAN_POINT('Ctrl Pts',(-0.493462957200432,-0.177024326825049,
1.0099536580922));
#33744=CARTESIAN_POINT('Ctrl Pts',(-0.511762781179148,-0.14429930310074,
1.00061845128527));
#33745=CARTESIAN_POINT('Ctrl Pts',(-0.529268075276157,-0.0928409665394226,
0.991396466802468));
#33746=CARTESIAN_POINT('Ctrl Pts',(-0.533501897135713,-0.0762225747374254,
0.989110885965947));
#33747=CARTESIAN_POINT('Ctrl Pts',(-0.536443649899848,-0.0595300000000001,
0.987512846410683));
#33748=CARTESIAN_POINT('',(-0.843383895613249,-0.05953,0.742736168477219));
#33749=CARTESIAN_POINT('Origin',(0.,-0.05953,0.));
#33750=CARTESIAN_POINT('',(-1.10653577764992,-0.05953,0.196295654879792));
#33751=CARTESIAN_POINT('Ctrl Pts',(-0.843383895613249,-0.0595300000000001,
0.742736168477219));
#33752=CARTESIAN_POINT('Ctrl Pts',(-0.84559647055299,-0.0762225747374255,
0.740223768851062));
#33753=CARTESIAN_POINT('Ctrl Pts',(-0.848766861100456,-0.0928409665394227,
0.736604687327351));
#33754=CARTESIAN_POINT('Ctrl Pts',(-0.861652925570091,-0.144299303100741,
0.721590372101268));
#33755=CARTESIAN_POINT('Ctrl Pts',(-0.87482617317514,-0.177024326825049,
0.705826641853758));
#33756=CARTESIAN_POINT('Ctrl Pts',(-0.902215926359523,-0.227269801620063,
0.670378702718353));
#33757=CARTESIAN_POINT('Ctrl Pts',(-0.919707509403859,-0.251265615809407,
0.646415841396062));
#33758=CARTESIAN_POINT('Ctrl Pts',(-0.947476448101718,-0.279889827963178,
0.604769294586516));
#33759=CARTESIAN_POINT('Ctrl Pts',(-0.961329858300736,-0.290879136862659,
0.582692035672022));
#33760=CARTESIAN_POINT('Ctrl Pts',(-0.988250837578047,-0.305251990234488,
0.535766169015486));
#33761=CARTESIAN_POINT('Ctrl Pts',(-1.00129756308006,-0.308638795020976,
0.510906605094603));
#33762=CARTESIAN_POINT('Ctrl Pts',(-1.02374168767024,-0.308638795020976,
0.46430090015576));
#33763=CARTESIAN_POINT('Ctrl Pts',(-1.03504317708586,-0.305251990234488,
0.438600874831839));
#33764=CARTESIAN_POINT('Ctrl Pts',(-1.05494634094458,-0.290879136862659,
0.388295406390235));
#33765=CARTESIAN_POINT('Ctrl Pts',(-1.06356957703048,-0.279889827963178,
0.363699428370917));
#33766=CARTESIAN_POINT('Ctrl Pts',(-1.0788165083757,-0.251265615809407,
0.316022600643821));
#33767=CARTESIAN_POINT('Ctrl Pts',(-1.08664560412098,-0.227269801620063,
0.287406530683752));
#33768=CARTESIAN_POINT('Ctrl Pts',(-1.09728268713976,-0.177024326825049,
0.243890930799337));
#33769=CARTESIAN_POINT('Ctrl Pts',(-1.10139388218929,-0.144299303100741,
0.22376314604679));
#33770=CARTESIAN_POINT('Ctrl Pts',(-1.10509821673782,-0.0928409665394227,
0.204327142733961));
#33771=CARTESIAN_POINT('Ctrl Pts',(-1.10595102243643,-0.0762225747374254,
0.199591971170104));
#33772=CARTESIAN_POINT('Ctrl Pts',(-1.10653577764992,-0.0595300000000001,
0.196295654879792));
#33773=CARTESIAN_POINT('',(-1.123812,-0.05953,1.37627276864339E-16));
#33774=CARTESIAN_POINT('Origin',(0.,-0.05953,0.));
#33775=CARTESIAN_POINT('',(-1.123812,-0.35718,1.37627276864339E-16));
#33776=CARTESIAN_POINT('',(-1.123812,-0.208355,1.37627276864339E-16));
#33777=CARTESIAN_POINT('Origin',(0.,-0.35718,0.));
#33778=CARTESIAN_POINT('',(-1.10653577764992,-0.05953,-0.196295654879793));
#33779=CARTESIAN_POINT('Origin',(0.,-0.05953,0.));
#33780=CARTESIAN_POINT('',(-0.843383895613249,-0.05953,-0.742736168477219));
#33781=CARTESIAN_POINT('Ctrl Pts',(-1.10653577764992,-0.0595300000000001,
-0.196295654879792));
#33782=CARTESIAN_POINT('Ctrl Pts',(-1.10595102243643,-0.0762225747374255,
-0.199591971170104));
#33783=CARTESIAN_POINT('Ctrl Pts',(-1.10509821673782,-0.0928409665394228,
-0.204327142733962));
#33784=CARTESIAN_POINT('Ctrl Pts',(-1.10139388218929,-0.144299303100741,
-0.22376314604679));
#33785=CARTESIAN_POINT('Ctrl Pts',(-1.09728268713976,-0.177024326825049,
-0.243890930799338));
#33786=CARTESIAN_POINT('Ctrl Pts',(-1.08664560412098,-0.227269801620063,
-0.287406530683753));
#33787=CARTESIAN_POINT('Ctrl Pts',(-1.0788165083757,-0.251265615809407,
-0.316022600643821));
#33788=CARTESIAN_POINT('Ctrl Pts',(-1.06356957703048,-0.279889827963178,
-0.363699428370918));
#33789=CARTESIAN_POINT('Ctrl Pts',(-1.05494634094458,-0.290879136862659,
-0.388295406390235));
#33790=CARTESIAN_POINT('Ctrl Pts',(-1.03504317708586,-0.305251990234488,
-0.438600874831839));
#33791=CARTESIAN_POINT('Ctrl Pts',(-1.02374168767024,-0.308638795020976,
-0.46430090015576));
#33792=CARTESIAN_POINT('Ctrl Pts',(-1.00129756308006,-0.308638795020976,
-0.510906605094603));
#33793=CARTESIAN_POINT('Ctrl Pts',(-0.988250837578047,-0.305251990234488,
-0.535766169015486));
#33794=CARTESIAN_POINT('Ctrl Pts',(-0.961329858300736,-0.290879136862659,
-0.582692035672022));
#33795=CARTESIAN_POINT('Ctrl Pts',(-0.947476448101718,-0.279889827963178,
-0.604769294586516));
#33796=CARTESIAN_POINT('Ctrl Pts',(-0.919707509403859,-0.251265615809407,
-0.646415841396062));
#33797=CARTESIAN_POINT('Ctrl Pts',(-0.902215926359523,-0.227269801620064,
-0.670378702718353));
#33798=CARTESIAN_POINT('Ctrl Pts',(-0.87482617317514,-0.177024326825049,
-0.705826641853758));
#33799=CARTESIAN_POINT('Ctrl Pts',(-0.861652925570091,-0.144299303100741,
-0.721590372101268));
#33800=CARTESIAN_POINT('Ctrl Pts',(-0.848766861100456,-0.0928409665394229,
-0.736604687327351));
#33801=CARTESIAN_POINT('Ctrl Pts',(-0.84559647055299,-0.0762225747374255,
-0.740223768851063));
#33802=CARTESIAN_POINT('Ctrl Pts',(-0.843383895613249,-0.0595300000000001,
-0.742736168477219));
#33803=CARTESIAN_POINT('',(-0.536443649899847,-0.05953,-0.987512846410683));
#33804=CARTESIAN_POINT('Origin',(0.,-0.05953,0.));
#33805=CARTESIAN_POINT('',(0.0548532617164172,-0.05953,-1.12247250791415));
#33806=CARTESIAN_POINT('Ctrl Pts',(-0.536443649899848,-0.0595300000000001,
-0.987512846410683));
#33807=CARTESIAN_POINT('Ctrl Pts',(-0.533501897135712,-0.0762225747374254,
-0.989110885965947));
#33808=CARTESIAN_POINT('Ctrl Pts',(-0.529268075276156,-0.0928409665394227,
-0.991396466802469));
#33809=CARTESIAN_POINT('Ctrl Pts',(-0.511762781179147,-0.144299303100741,
-1.00061845128527));
#33810=CARTESIAN_POINT('Ctrl Pts',(-0.493462957200432,-0.177024326825049,
-1.0099536580922));
#33811=CARTESIAN_POINT('Ctrl Pts',(-0.45280897844858,-0.227269801620063,
-1.02876878445619));
#33812=CARTESIAN_POINT('Ctrl Pts',(-0.425554672694337,-0.251265615809407,
-1.04048957871266));
#33813=CARTESIAN_POINT('Ctrl Pts',(-0.3787731215897,-0.279889827963178,
-1.05829506364875));
#33814=CARTESIAN_POINT('Ctrl Pts',(-0.354166711873529,-0.290879136862659,
-1.06688848765783));
#33815=CARTESIAN_POINT('Ctrl Pts',(-0.302426893214944,-0.305251990234488,
-1.08269251410343));
#33816=CARTESIAN_POINT('Ctrl Pts',(-0.275287440920027,-0.308638795020976,
-1.0898803575765));
#33817=CARTESIAN_POINT('Ctrl Pts',(-0.224855950742601,-0.308638795020976,
-1.10139101611326));
#33818=CARTESIAN_POINT('Ctrl Pts',(-0.19728546073067,-0.305251990234488,
-1.10669035995599));
#33819=CARTESIAN_POINT('Ctrl Pts',(-0.143812384801039,-0.290879136862659,
-1.11490049012186));
#33820=CARTESIAN_POINT('Ctrl Pts',(-0.117914228755037,-0.279889827963178,
-1.1178344036749));
#33821=CARTESIAN_POINT('Ctrl Pts',(-0.0680399972366989,-0.251265615809407,
-1.12208997038458));
#33822=CARTESIAN_POINT('Ctrl Pts',(-0.0383992541984084,-0.227269801620063,
-1.12335509974011));
#33823=CARTESIAN_POINT('Ctrl Pts',(0.00639229239215326,-0.177024326825049,
-1.12404235695137));
#33824=CARTESIAN_POINT('Ctrl Pts',(0.0269302585198977,-0.144299303100741,
-1.12357162229597));
#33825=CARTESIAN_POINT('Ctrl Pts',(0.04670325263426,-0.0928409665394228,
-1.12285816383385));
#33826=CARTESIAN_POINT('Ctrl Pts',(0.0515094706813703,-0.0762225747374255,
-1.12263591311425));
#33827=CARTESIAN_POINT('Ctrl Pts',(0.0548532617164176,-0.0595300000000001,
-1.12247250791414));
#33828=CARTESIAN_POINT('',(0.437601487681057,-0.05953,-1.03511272300331));
#33829=CARTESIAN_POINT('Origin',(0.,-0.05953,0.));
#33830=CARTESIAN_POINT('',(0.911784794170997,-0.05953,-0.656964154625313));
#33831=CARTESIAN_POINT('Ctrl Pts',(0.437601487681056,-0.0595300000000001,
-1.03511272300331));
#33832=CARTESIAN_POINT('Ctrl Pts',(0.440685038163619,-0.0762225747374255,
-1.03380912944435));
#33833=CARTESIAN_POINT('Ctrl Pts',(0.445111721969657,-0.0928409665394228,
-1.03192403056628));
#33834=CARTESIAN_POINT('Ctrl Pts',(0.463236132117164,-0.144299303100741,
-1.0239876538093));
#33835=CARTESIAN_POINT('Ctrl Pts',(0.481944444320713,-0.177024326825049,
-1.01550068154148));
#33836=CARTESIAN_POINT('Ctrl Pts',(0.522002043615455,-0.227269801620064,
-0.995447160474328));
#33837=CARTESIAN_POINT('Ctrl Pts',(0.548158511259203,-0.251265615809407,
-0.981446681891443));
#33838=CARTESIAN_POINT('Ctrl Pts',(0.591247219971725,-0.279889827963178,
-0.955972930713954));
#33839=CARTESIAN_POINT('Ctrl Pts',(0.613307674922609,-0.290879136862659,
-0.942092777160053));
#33840=CARTESIAN_POINT('Ctrl Pts',(0.657923009631182,-0.305251990234487,
-0.91149460735272));
#33841=CARTESIAN_POINT('Ctrl Pts',(0.680463863683393,-0.308638795020976,
-0.894757676234429));
#33842=CARTESIAN_POINT('Ctrl Pts',(0.720906778729542,-0.308638795020976,
-0.862505527716294));
#33843=CARTESIAN_POINT('Ctrl Pts',(0.742239891936899,-0.305251990234488,
-0.844254137480381));
#33844=CARTESIAN_POINT('Ctrl Pts',(0.781998747691872,-0.290879136862659,
-0.80756613568454));
#33845=CARTESIAN_POINT('Ctrl Pts',(0.800439809856112,-0.279889827963178,
-0.789147407129765));
#33846=CARTESIAN_POINT('Ctrl Pts',(0.834863020612702,-0.251265615809407,
-0.752807465209441));
#33847=CARTESIAN_POINT('Ctrl Pts',(0.854332839576145,-0.227269801620064,
-0.73042219438957));
#33848=CARTESIAN_POINT('Ctrl Pts',(0.882797231409153,-0.177024326825049,
-0.695831250979106));
#33849=CARTESIAN_POINT('Ctrl Pts',(0.895234408667242,-0.144299303100741,
-0.679480524217551));
#33850=CARTESIAN_POINT('Ctrl Pts',(0.907004864562642,-0.0928409665394228,
-0.663576540841106));
#33851=CARTESIAN_POINT('Ctrl Pts',(0.909827729890942,-0.0762225747374256,
-0.659680317203144));
#33852=CARTESIAN_POINT('Ctrl Pts',(0.911784794170998,-0.0595300000000001,
-0.656964154625312));
#33853=CARTESIAN_POINT('',(1.08212377959455,-0.05953,-0.303251606722892));
#33854=CARTESIAN_POINT('Origin',(0.,-0.05953,0.));
#33855=CARTESIAN_POINT('',(1.08212377959455,-0.05953,0.303251606722892));
#33856=CARTESIAN_POINT('Ctrl Pts',(1.08212377959455,-0.0595300000000001,
-0.303251606722892));
#33857=CARTESIAN_POINT('Ctrl Pts',(1.0830271513892,-0.0762225747374255,
-0.300028012588062));
#33858=CARTESIAN_POINT('Ctrl Pts',(1.08431331394788,-0.0928409665394228,
-0.2953917518996));
#33859=CARTESIAN_POINT('Ctrl Pts',(1.08940878963422,-0.144299303100741,
-0.276273267473431));
#33860=CARTESIAN_POINT('Ctrl Pts',(1.09443784939331,-0.177024326825049,
-0.256354979351213));
#33861=CARTESIAN_POINT('Ctrl Pts',(1.10373487993589,-0.227269801620064,
-0.212533521233765));
#33862=CARTESIAN_POINT('Ctrl Pts',(1.10909715583869,-0.251265615809407,
-0.183354415742157));
#33863=CARTESIAN_POINT('Ctrl Pts',(1.1160463456491,-0.279889827963178,-0.133783682657561));
#33864=CARTESIAN_POINT('Ctrl Pts',(1.11894887330541,-0.290879136862659,
-0.107881990270302));
#33865=CARTESIAN_POINT('Ctrl Pts',(1.12284346704144,-0.305251990234488,
-0.0539226701638766));
#33866=CARTESIAN_POINT('Ctrl Pts',(1.123812,-0.308638795020976,-0.025864214957475));
#33867=CARTESIAN_POINT('Ctrl Pts',(1.123812,-0.308638795020976,0.025864214957475));
#33868=CARTESIAN_POINT('Ctrl Pts',(1.12284346704144,-0.305251990234488,
0.0539226701638766));
#33869=CARTESIAN_POINT('Ctrl Pts',(1.11894887330541,-0.290879136862659,
0.107881990270302));
#33870=CARTESIAN_POINT('Ctrl Pts',(1.1160463456491,-0.279889827963178,0.133783682657561));
#33871=CARTESIAN_POINT('Ctrl Pts',(1.10909715583869,-0.251265615809407,
0.183354415742157));
#33872=CARTESIAN_POINT('Ctrl Pts',(1.10373487993589,-0.227269801620064,
0.212533521233765));
#33873=CARTESIAN_POINT('Ctrl Pts',(1.09443784939331,-0.177024326825049,
0.256354979351213));
#33874=CARTESIAN_POINT('Ctrl Pts',(1.08940878963422,-0.144299303100741,
0.276273267473431));
#33875=CARTESIAN_POINT('Ctrl Pts',(1.08431331394788,-0.0928409665394228,
0.2953917518996));
#33876=CARTESIAN_POINT('Ctrl Pts',(1.0830271513892,-0.0762225747374255,
0.300028012588062));
#33877=CARTESIAN_POINT('Ctrl Pts',(1.08212377959455,-0.0595300000000001,
0.303251606722892));
#33878=CARTESIAN_POINT('Origin',(0.,-0.05953,0.));
#33879=CARTESIAN_POINT('Origin',(0.,-0.05953,0.));
#33880=CARTESIAN_POINT('',(0.0589974094846122,-0.05953,1.07456964270265));
#33881=CARTESIAN_POINT('Origin',(0.,-0.05953,0.));
#33882=CARTESIAN_POINT('Origin',(-0.244773027351946,-0.05953,1.07242070340001));
#33883=CARTESIAN_POINT('Origin',(-0.244773027351946,0.,1.07242070340001));
#33884=CARTESIAN_POINT('',(-0.519393123750572,-0.05953,0.942555777842682));
#33885=CARTESIAN_POINT('Ctrl Pts',(-0.519393123750572,-0.05953,0.942555777842682));
#33886=CARTESIAN_POINT('Ctrl Pts',(-0.513714466572041,-0.0925528133349865,
0.945684988399766));
#33887=CARTESIAN_POINT('Ctrl Pts',(-0.503136848051455,-0.124911173756694,
0.951483858396181));
#33888=CARTESIAN_POINT('Ctrl Pts',(-0.47593627990192,-0.177924977804098,
0.965323333309091));
#33889=CARTESIAN_POINT('Ctrl Pts',(-0.460931856495794,-0.199697230012983,
0.972669835243841));
#33890=CARTESIAN_POINT('Ctrl Pts',(-0.426157505475872,-0.237895043532788,
0.988400002689705));
#33891=CARTESIAN_POINT('Ctrl Pts',(-0.406380688682952,-0.254319232363049,
0.996771768218699));
#33892=CARTESIAN_POINT('Ctrl Pts',(-0.364750145543744,-0.28018331644634,
1.01272583306292));
#33893=CARTESIAN_POINT('Ctrl Pts',(-0.340838910881557,-0.29104845371857,
1.02112815447116));
#33894=CARTESIAN_POINT('Ctrl Pts',(-0.290495481564827,-0.30527573347708,
1.036574285215));
#33895=CARTESIAN_POINT('Ctrl Pts',(-0.264056468041074,-0.308638795020976,
1.04359501395068));
#33896=CARTESIAN_POINT('Ctrl Pts',(-0.214892249704082,-0.308638795020976,
1.05481642595959));
#33897=CARTESIAN_POINT('Ctrl Pts',(-0.188025341585962,-0.30527573347708,
1.05996242598502));
#33898=CARTESIAN_POINT('Ctrl Pts',(-0.135965654106109,-0.29104845371857,
1.06788913840721));
#33899=CARTESIAN_POINT('Ctrl Pts',(-0.110776745452494,-0.28018331644634,
1.07069360430242));
#33900=CARTESIAN_POINT('Ctrl Pts',(-0.0663467128214646,-0.254319232363049,
1.07438230428002));
#33901=CARTESIAN_POINT('Ctrl Pts',(-0.0448960436540983,-0.237895043532788,
1.07542044338697));
#33902=CARTESIAN_POINT('Ctrl Pts',(-0.00674037211528124,-0.199697230012983,
1.07633607767727));
#33903=CARTESIAN_POINT('Ctrl Pts',(0.00996567398334777,-0.177924977804098,
1.07622728347683));
#33904=CARTESIAN_POINT('Ctrl Pts',(0.0404772621979741,-0.124911173756694,
1.07556023164702));
#33905=CARTESIAN_POINT('Ctrl Pts',(0.0525234025782719,-0.0925528133349865,
1.07492508698591));
#33906=CARTESIAN_POINT('Ctrl Pts',(0.0589974094846124,-0.05953,1.07456964270265));
#33907=CARTESIAN_POINT('Origin',(-0.244773027351946,-0.05953,1.07242070340001));
#33908=CARTESIAN_POINT('Origin',(0.,-0.05953,0.));
#33909=CARTESIAN_POINT('',(-0.803348093619616,-0.05953,0.716109245731214));
#33910=CARTESIAN_POINT('Origin',(0.,-0.05953,0.));
#33911=CARTESIAN_POINT('Origin',(-0.991065754692661,-0.05953,0.477272113029314));
#33912=CARTESIAN_POINT('Origin',(-0.991065754692661,0.,0.477272113029314));
#33913=CARTESIAN_POINT('',(-1.06075609691358,-0.05953,0.181596019242328));
#33914=CARTESIAN_POINT('Ctrl Pts',(-1.06075609691358,-0.05953,0.181596019242328));
#33915=CARTESIAN_POINT('Ctrl Pts',(-1.05966202740332,-0.0925528133349865,
0.187986803072856));
#33916=CARTESIAN_POINT('Ctrl Pts',(-1.05760072925372,-0.124911173756694,
0.199872254546857));
#33917=CARTESIAN_POINT('Ctrl Pts',(-1.05146158959546,-0.177924977804098,
0.22976728653846));
#33918=CARTESIAN_POINT('Ctrl Pts',(-1.04785021111757,-0.199697230012983,
0.246078686169301));
#33919=CARTESIAN_POINT('Ctrl Pts',(-1.03846709802406,-0.237895043532788,
0.283073967563097));
#33920=CARTESIAN_POINT('Ctrl Pts',(-1.03268176429485,-0.254319232363049,
0.303755815985685));
#33921=CARTESIAN_POINT('Ctrl Pts',(-1.01919893537026,-0.28018331644634,
0.346251081972725));
#33922=CARTESIAN_POINT('Ctrl Pts',(-1.01085972381132,-0.29104845371857,
0.370184399726282));
#33923=CARTESIAN_POINT('Ctrl Pts',(-0.99154738033959,-0.30527573347708,
0.419174982698463));
#33924=CARTESIAN_POINT('Ctrl Pts',(-0.980551951791748,-0.308638795020976,
0.444223188605045));
#33925=CARTESIAN_POINT('Ctrl Pts',(-0.958671816228589,-0.308638795020976,
0.489657758261848));
#33926=CARTESIAN_POINT('Ctrl Pts',(-0.945943877838127,-0.30527573347708,
0.51387163140139));
#33927=CARTESIAN_POINT('Ctrl Pts',(-0.91968254693063,-0.29104845371857,
0.559515758398093));
#33928=CARTESIAN_POINT('Ctrl Pts',(-0.906170138993533,-0.28018331644634,
0.580957796077825));
#33929=CARTESIAN_POINT('Ctrl Pts',(-0.8813524085237,-0.254319232363049,
0.617994461173994));
#33930=CARTESIAN_POINT('Ctrl Pts',(-0.868789784891799,-0.237895043532788,
0.635412538795143));
#33931=CARTESIAN_POINT('Ctrl Pts',(-0.845715984518854,-0.199697230012983,
0.66581473268113));
#33932=CARTESIAN_POINT('Ctrl Pts',(-0.835214876415962,-0.177924977804098,
0.678808213394124));
#33933=CARTESIAN_POINT('Ctrl Pts',(-0.815669690204649,-0.124911173756694,
0.702247233627224));
#33934=CARTESIAN_POINT('Ctrl Pts',(-0.807662468433796,-0.0925528133349865,
0.711269279199861));
#33935=CARTESIAN_POINT('Ctrl Pts',(-0.803348093619616,-0.05953,0.716109245731214));
#33936=CARTESIAN_POINT('Origin',(-0.991065754692661,-0.05953,0.477272113029314));
#33937=CARTESIAN_POINT('Origin',(0.,-0.05953,0.));
#33938=CARTESIAN_POINT('',(-1.076188,-0.05953,1.31795018948079E-16));
#33939=CARTESIAN_POINT('Origin',(0.,-0.05953,0.));
#33940=CARTESIAN_POINT('',(-1.06075609691358,-0.05953,-0.181596019242328));
#33941=CARTESIAN_POINT('Origin',(0.,-0.05953,0.));
#33942=CARTESIAN_POINT('Origin',(-0.991065754692661,-0.05953,-0.477272113029314));
#33943=CARTESIAN_POINT('Origin',(-0.991065754692661,0.,-0.477272113029314));
#33944=CARTESIAN_POINT('',(-0.803348093619616,-0.05953,-0.716109245731215));
#33945=CARTESIAN_POINT('Ctrl Pts',(-0.803348093619616,-0.05953,-0.716109245731215));
#33946=CARTESIAN_POINT('Ctrl Pts',(-0.807662468433795,-0.0925528133349865,
-0.711269279199862));
#33947=CARTESIAN_POINT('Ctrl Pts',(-0.815669690204649,-0.124911173756694,
-0.702247233627224));
#33948=CARTESIAN_POINT('Ctrl Pts',(-0.835214876415962,-0.177924977804098,
-0.678808213394124));
#33949=CARTESIAN_POINT('Ctrl Pts',(-0.845715984518854,-0.199697230012983,
-0.66581473268113));
#33950=CARTESIAN_POINT('Ctrl Pts',(-0.868789784891799,-0.237895043532788,
-0.635412538795143));
#33951=CARTESIAN_POINT('Ctrl Pts',(-0.8813524085237,-0.254319232363049,
-0.617994461173994));
#33952=CARTESIAN_POINT('Ctrl Pts',(-0.906170138993533,-0.28018331644634,
-0.580957796077826));
#33953=CARTESIAN_POINT('Ctrl Pts',(-0.91968254693063,-0.29104845371857,
-0.559515758398093));
#33954=CARTESIAN_POINT('Ctrl Pts',(-0.945943877838127,-0.30527573347708,
-0.51387163140139));
#33955=CARTESIAN_POINT('Ctrl Pts',(-0.958671816228589,-0.308638795020976,
-0.489657758261848));
#33956=CARTESIAN_POINT('Ctrl Pts',(-0.980551951791748,-0.308638795020976,
-0.444223188605045));
#33957=CARTESIAN_POINT('Ctrl Pts',(-0.99154738033959,-0.30527573347708,
-0.419174982698463));
#33958=CARTESIAN_POINT('Ctrl Pts',(-1.01085972381132,-0.29104845371857,
-0.370184399726282));
#33959=CARTESIAN_POINT('Ctrl Pts',(-1.01919893537026,-0.28018331644634,
-0.346251081972725));
#33960=CARTESIAN_POINT('Ctrl Pts',(-1.03268176429485,-0.254319232363049,
-0.303755815985685));
#33961=CARTESIAN_POINT('Ctrl Pts',(-1.03846709802406,-0.237895043532788,
-0.283073967563097));
#33962=CARTESIAN_POINT('Ctrl Pts',(-1.04785021111757,-0.199697230012983,
-0.246078686169302));
#33963=CARTESIAN_POINT('Ctrl Pts',(-1.05146158959546,-0.177924977804098,
-0.229767286538461));
#33964=CARTESIAN_POINT('Ctrl Pts',(-1.05760072925372,-0.124911173756694,
-0.199872254546858));
#33965=CARTESIAN_POINT('Ctrl Pts',(-1.05966202740332,-0.0925528133349864,
-0.187986803072857));
#33966=CARTESIAN_POINT('Ctrl Pts',(-1.06075609691358,-0.05953,-0.181596019242328));
#33967=CARTESIAN_POINT('Origin',(-0.991065754692661,-0.05953,-0.477272113029314));
#33968=CARTESIAN_POINT('Origin',(0.,-0.05953,0.));
#33969=CARTESIAN_POINT('',(-0.519393123750572,-0.05953,-0.942555777842682));
#33970=CARTESIAN_POINT('Origin',(0.,-0.05953,0.));
#33971=CARTESIAN_POINT('Origin',(-0.244773027351946,-0.05953,-1.07242070340001));
#33972=CARTESIAN_POINT('Origin',(-0.244773027351946,0.,-1.07242070340001));
#33973=CARTESIAN_POINT('',(0.0589974094846125,-0.05953,-1.07456964270265));
#33974=CARTESIAN_POINT('Ctrl Pts',(0.0589974094846127,-0.05953,-1.07456964270265));
#33975=CARTESIAN_POINT('Ctrl Pts',(0.0525234025782722,-0.0925528133349865,
-1.07492508698591));
#33976=CARTESIAN_POINT('Ctrl Pts',(0.0404772621979744,-0.124911173756694,
-1.07556023164702));
#33977=CARTESIAN_POINT('Ctrl Pts',(0.0099656739833481,-0.177924977804098,
-1.07622728347683));
#33978=CARTESIAN_POINT('Ctrl Pts',(-0.00674037211528096,-0.199697230012983,
-1.07633607767727));
#33979=CARTESIAN_POINT('Ctrl Pts',(-0.044896043654098,-0.237895043532788,
-1.07542044338697));
#33980=CARTESIAN_POINT('Ctrl Pts',(-0.0663467128214644,-0.254319232363049,
-1.07438230428002));
#33981=CARTESIAN_POINT('Ctrl Pts',(-0.110776745452493,-0.28018331644634,
-1.07069360430242));
#33982=CARTESIAN_POINT('Ctrl Pts',(-0.135965654106109,-0.29104845371857,
-1.06788913840721));
#33983=CARTESIAN_POINT('Ctrl Pts',(-0.188025341585962,-0.30527573347708,
-1.05996242598502));
#33984=CARTESIAN_POINT('Ctrl Pts',(-0.214892249704082,-0.308638795020976,
-1.05481642595959));
#33985=CARTESIAN_POINT('Ctrl Pts',(-0.264056468041074,-0.308638795020976,
-1.04359501395068));
#33986=CARTESIAN_POINT('Ctrl Pts',(-0.290495481564827,-0.30527573347708,
-1.036574285215));
#33987=CARTESIAN_POINT('Ctrl Pts',(-0.340838910881557,-0.291048453718569,
-1.02112815447116));
#33988=CARTESIAN_POINT('Ctrl Pts',(-0.364750145543744,-0.28018331644634,
-1.01272583306292));
#33989=CARTESIAN_POINT('Ctrl Pts',(-0.406380688682952,-0.254319232363049,
-0.996771768218699));
#33990=CARTESIAN_POINT('Ctrl Pts',(-0.426157505475872,-0.237895043532788,
-0.988400002689705));
#33991=CARTESIAN_POINT('Ctrl Pts',(-0.460931856495794,-0.199697230012983,
-0.972669835243841));
#33992=CARTESIAN_POINT('Ctrl Pts',(-0.475936279901919,-0.177924977804098,
-0.965323333309091));
#33993=CARTESIAN_POINT('Ctrl Pts',(-0.503136848051454,-0.124911173756694,
-0.951483858396181));
#33994=CARTESIAN_POINT('Ctrl Pts',(-0.513714466572041,-0.0925528133349865,
-0.945684988399766));
#33995=CARTESIAN_POINT('Ctrl Pts',(-0.519393123750572,-0.05953,-0.942555777842682));
#33996=CARTESIAN_POINT('Origin',(-0.244773027351946,-0.05953,-1.07242070340001));
#33997=CARTESIAN_POINT('Origin',(0.,-0.05953,0.));
#33998=CARTESIAN_POINT('',(0.413083465285518,-0.05953,-0.993751811093549));
#33999=CARTESIAN_POINT('Origin',(0.,-0.05953,0.));
#34000=CARTESIAN_POINT('Origin',(0.685838782044607,-0.05953,-0.860014630714833));
#34001=CARTESIAN_POINT('Origin',(0.685838782044607,0.,-0.860014630714833));
#34002=CARTESIAN_POINT('',(0.876916659919095,-0.05953,-0.623857181492959));
#34003=CARTESIAN_POINT('Ctrl Pts',(0.876916659919095,-0.05953,-0.623857181492958));
#34004=CARTESIAN_POINT('Ctrl Pts',(0.873158080166742,-0.0925528133349865,
-0.62914037979579));
#34005=CARTESIAN_POINT('Ctrl Pts',(0.866144010579847,-0.124911173756694,
-0.638954437806245));
#34006=CARTESIAN_POINT('Ctrl Pts',(0.847641868610495,-0.177924977804098,
-0.663225258065736));
#34007=CARTESIAN_POINT('Ctrl Pts',(0.837310877969633,-0.199697230012983,
-0.676354402927683));
#34008=CARTESIAN_POINT('Ctrl Pts',(0.81280533416753,-0.237895043532788,
-0.705614819529209));
#34009=CARTESIAN_POINT('Ctrl Pts',(0.798619410861634,-0.254319232363049,
-0.721738358858166));
#34010=CARTESIAN_POINT('Ctrl Pts',(0.768033796848072,-0.28018331644634,
-0.754175290318038));
#34011=CARTESIAN_POINT('Ctrl Pts',(0.750136149454208,-0.29104845371857,
-0.772120216227122));
#34012=CARTESIAN_POINT('Ctrl Pts',(0.711480111898423,-0.30527573347708,
-0.807879894508811));
#34013=CARTESIAN_POINT('Ctrl Pts',(0.690705563850638,-0.308638795020976,
-0.825676810575913));
#34014=CARTESIAN_POINT('Ctrl Pts',(0.651278921914856,-0.308638795020976,
-0.857118508332695));
#34015=CARTESIAN_POINT('Ctrl Pts',(0.629305439856167,-0.30527573347708,
-0.873412008702649));
#34016=CARTESIAN_POINT('Ctrl Pts',(0.585840553788742,-0.29104845371857,
-0.903141581680914));
#34017=CARTESIAN_POINT('Ctrl Pts',(0.564362943424239,-0.28018331644634,
-0.916597376014514));
#34018=CARTESIAN_POINT('Ctrl Pts',(0.525933334162556,-0.254319232363049,
-0.939198248544427));
#34019=CARTESIAN_POINT('Ctrl Pts',(0.507057380724533,-0.237895043532788,
-0.949440676105255));
#34020=CARTESIAN_POINT('Ctrl Pts',(0.473077587363686,-0.199697230012983,
-0.966820759530997));
#34021=CARTESIAN_POINT('Ctrl Pts',(0.457978755888596,-0.177924977804098,
-0.973971221090534));
#34022=CARTESIAN_POINT('Ctrl Pts',(0.430199341854858,-0.124911173756694,
-0.986608710139579));
#34023=CARTESIAN_POINT('Ctrl Pts',(0.419070565453384,-0.0925528133349865,
-0.991263089003441));
#34024=CARTESIAN_POINT('Ctrl Pts',(0.413083465285518,-0.05953,-0.993751811093549));
#34025=CARTESIAN_POINT('Origin',(0.685838782044607,-0.05953,-0.860014630714833));
#34026=CARTESIAN_POINT('Origin',(0.,-0.208355,0.));
#34027=CARTESIAN_POINT('',(-1.076188,-0.35718,1.31795018948079E-16));
#34028=CARTESIAN_POINT('Origin',(0.,-0.35718,0.));
#34029=CARTESIAN_POINT('',(-1.076188,-0.208355,1.31795018948079E-16));
#34030=CARTESIAN_POINT('',(1.03449977959455,-0.05953,0.296632461748266));
#34031=CARTESIAN_POINT('Origin',(0.,-0.05953,0.));
#34032=CARTESIAN_POINT('',(1.03449977959455,-0.05953,-0.296632461748266));
#34033=CARTESIAN_POINT('Ctrl Pts',(1.03449977959455,-0.05953,0.296632461748267));
#34034=CARTESIAN_POINT('Ctrl Pts',(1.03628691421076,-0.0925528133349865,
0.290399865505497));
#34035=CARTESIAN_POINT('Ctrl Pts',(1.03958665287714,-0.124911173756694,
0.278797079997872));
#34036=CARTESIAN_POINT('Ctrl Pts',(1.0470264474309,-0.177924977804098,0.249198913998601));
#34037=CARTESIAN_POINT('Ctrl Pts',(1.05084995891418,-0.199697230012983,
0.232935932341942));
#34038=CARTESIAN_POINT('Ctrl Pts',(1.05844771715377,-0.237895043532788,
0.195533155353269));
#34039=CARTESIAN_POINT('Ctrl Pts',(1.06220882929878,-0.254319232363049,
0.17438929156337));
#34040=CARTESIAN_POINT('Ctrl Pts',(1.06849922508772,-0.28018331644634,0.130252399648131));
#34041=CARTESIAN_POINT('Ctrl Pts',(1.07137013248666,-0.29104845371857,0.105070977154072));
#34042=CARTESIAN_POINT('Ctrl Pts',(1.07522652957392,-0.30527573347708,0.0525526752791107));
#34043=CARTESIAN_POINT('Ctrl Pts',(1.076188,-0.308638795020976,0.025214283908933));
#34044=CARTESIAN_POINT('Ctrl Pts',(1.076188,-0.308638795020976,-0.025214283908933));
#34045=CARTESIAN_POINT('Ctrl Pts',(1.07522652957392,-0.30527573347708,-0.0525526752791107));
#34046=CARTESIAN_POINT('Ctrl Pts',(1.07137013248666,-0.29104845371857,-0.105070977154072));
#34047=CARTESIAN_POINT('Ctrl Pts',(1.06849922508772,-0.28018331644634,-0.130252399648131));
#34048=CARTESIAN_POINT('Ctrl Pts',(1.06220882929878,-0.254319232363049,
-0.17438929156337));
#34049=CARTESIAN_POINT('Ctrl Pts',(1.05844771715377,-0.237895043532788,
-0.195533155353269));
#34050=CARTESIAN_POINT('Ctrl Pts',(1.05084995891418,-0.199697230012983,
-0.232935932341942));
#34051=CARTESIAN_POINT('Ctrl Pts',(1.0470264474309,-0.177924977804098,-0.249198913998601));
#34052=CARTESIAN_POINT('Ctrl Pts',(1.03958665287714,-0.124911173756694,
-0.278797079997872));
#34053=CARTESIAN_POINT('Ctrl Pts',(1.03628691421076,-0.0925528133349865,
-0.290399865505497));
#34054=CARTESIAN_POINT('Ctrl Pts',(1.03449977959455,-0.05953,-0.296632461748267));
#34055=CARTESIAN_POINT('Origin',(0.,-0.05953,0.));
#34056=CARTESIAN_POINT('Origin',(0.,-0.05953,0.));
#34057=CARTESIAN_POINT('Origin',(1.1,-0.05953,0.));
#34058=CARTESIAN_POINT('Origin',(1.1,0.,0.));
#34059=CARTESIAN_POINT('Origin',(1.1,-0.05953,0.));
#34060=CARTESIAN_POINT('Origin',(0.,-0.35718,0.));
#34061=CARTESIAN_POINT('Origin',(0.,-0.05953,0.));
#62805=UNCERTAINTY_MEASURE_WITH_UNIT(LENGTH_MEASURE(0.001),#62985,
'DISTANCE_ACCURACY_VALUE',
'Maximum model space distance between geometric entities at asserted c
onnectivities');
#62885=UNCERTAINTY_MEASURE_WITH_UNIT(LENGTH_MEASURE(0.001),#62985,
'DISTANCE_ACCURACY_VALUE',
'Maximum model space distance between geometric entities at asserted c
onnectivities');
#62904=(
GEOMETRIC_REPRESENTATION_CONTEXT(3)
GLOBAL_UNCERTAINTY_ASSIGNED_CONTEXT((#62805))
GLOBAL_UNIT_ASSIGNED_CONTEXT((#62985,#62987,#62988))
REPRESENTATION_CONTEXT('','3D')
);
#62984=(
GEOMETRIC_REPRESENTATION_CONTEXT(3)
GLOBAL_UNCERTAINTY_ASSIGNED_CONTEXT((#62885))
GLOBAL_UNIT_ASSIGNED_CONTEXT((#62985,#62987,#62988))
REPRESENTATION_CONTEXT('','3D')
);
#62985=(
LENGTH_UNIT()
NAMED_UNIT(*)
SI_UNIT(.CENTI.,.METRE.)
);
#62987=(
NAMED_UNIT(*)
PLANE_ANGLE_UNIT()
SI_UNIT($,.RADIAN.)
);
#62988=(
NAMED_UNIT(*)
SI_UNIT($,.STERADIAN.)
SOLID_ANGLE_UNIT()
);
#63007=SHAPE_DEFINITION_REPRESENTATION(#63105,#63367);
#63105=PRODUCT_DEFINITION_SHAPE('',$,#63466);
#63367=SHAPE_REPRESENTATION('',(#24341),#62904);
#63447=PRODUCT_DEFINITION_CONTEXT('part definition',#63743,'design');
#63466=PRODUCT_DEFINITION('Cage','Cage',#63564,#63447);
#63564=PRODUCT_DEFINITION_FORMATION('',$,#63763);
#63743=APPLICATION_CONTEXT(
'Core Data for Automotive Mechanical Design Process');
#63744=PRODUCT_CONTEXT('part definition',#63743,'mechanical');
#63763=PRODUCT('Cage','Cage','Cage',(#63744));
#63906=COLOUR_RGB('Grey',0.48,0.52,0.57);
#63907=FILL_AREA_STYLE_COLOUR('',#63906);
#63908=FILL_AREA_STYLE('',(#63907));
#63909=SURFACE_STYLE_FILL_AREA(#63908);
#63910=SURFACE_SIDE_STYLE('',(#63909));
#63911=SURFACE_STYLE_USAGE(.BOTH.,#63910);
#63912=PRESENTATION_STYLE_ASSIGNMENT((#63911));
ENDSEC;
END-ISO-10303-21;
